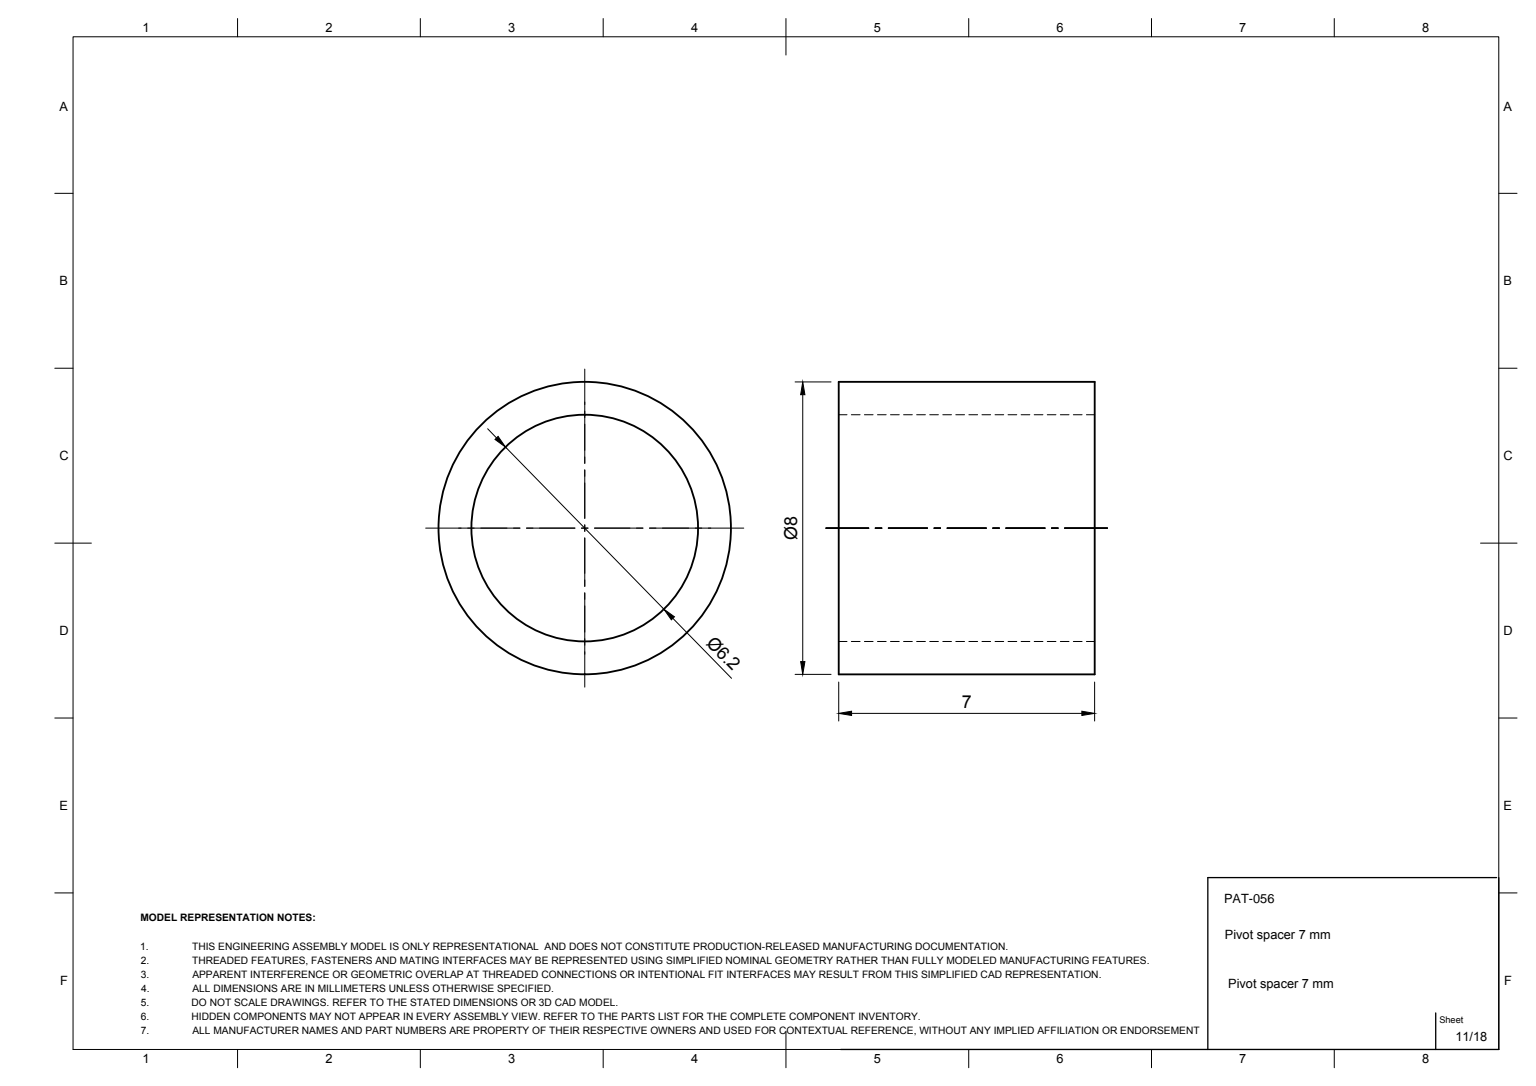
ISO-10303-21;
HEADER;
/* Generated by software containing ST-Developer
 * from STEP Tools, Inc. (www.steptools.com) 
 */

FILE_DESCRIPTION(
/* description */ ('Hook toggle clamp'),
/* implementation_level */ '2;1');

FILE_NAME(
/* name */ 'Pivot spacer 7 mm.step',
/* time_stamp */ '2026-10-27T21:56:56-07:00',
/* author */ (''),
/* organization */ (''),
/* preprocessor_version */ 'ST-DEVELOPER v20.2',
/* originating_system */ 'Autodesk Translation Framework v15.17.0.0',
/* authorisation */ '');

FILE_SCHEMA (('AUTOMOTIVE_DESIGN { 1 0 10303 214 3 1 1 }'));
ENDSEC;

DATA;
#10=MECHANICAL_DESIGN_GEOMETRIC_PRESENTATION_REPRESENTATION('',(#194),#5458);
#160=SHAPE_REPRESENTATION_RELATIONSHIP('SRR','None',#5542,#177);
#177=ADVANCED_BREP_SHAPE_REPRESENTATION('',(#211),#5444);
#194=STYLED_ITEM('',(#5703),#211);
#211=MANIFOLD_SOLID_BREP('Body1',#2975);
#251=FACE_BOUND('',#676,.T.);
#252=FACE_BOUND('',#678,.T.);
#336=PLANE('',#3312);
#337=PLANE('',#3313);
#471=FACE_OUTER_BOUND('',#673,.T.);
#472=FACE_OUTER_BOUND('',#674,.T.);
#473=FACE_OUTER_BOUND('',#675,.T.);
#474=FACE_OUTER_BOUND('',#677,.T.);
#673=EDGE_LOOP('',(#2377,#2378,#2379,#2380));
#674=EDGE_LOOP('',(#2381,#2382,#2383,#2384));
#675=EDGE_LOOP('',(#2385));
#676=EDGE_LOOP('',(#2386));
#677=EDGE_LOOP('',(#2387));
#678=EDGE_LOOP('',(#2388));
#934=LINE('',#4834,#1171);
#935=LINE('',#4840,#1172);
#1171=VECTOR('',#3914,0.31);
#1172=VECTOR('',#3921,0.4);
#1312=CIRCLE('',#3307,0.31);
#1313=CIRCLE('',#3308,0.31);
#1314=CIRCLE('',#3310,0.4);
#1315=CIRCLE('',#3311,0.4);
#1507=VERTEX_POINT('',#4831);
#1508=VERTEX_POINT('',#4833);
#1509=VERTEX_POINT('',#4837);
#1510=VERTEX_POINT('',#4839);
#1815=EDGE_CURVE('',#1507,#1507,#1312,.T.);
#1816=EDGE_CURVE('',#1507,#1508,#934,.T.);
#1817=EDGE_CURVE('',#1508,#1508,#1313,.T.);
#1818=EDGE_CURVE('',#1509,#1509,#1314,.T.);
#1819=EDGE_CURVE('',#1509,#1510,#935,.T.);
#1820=EDGE_CURVE('',#1510,#1510,#1315,.T.);
#2377=ORIENTED_EDGE('',*,*,#1815,.F.);
#2378=ORIENTED_EDGE('',*,*,#1816,.T.);
#2379=ORIENTED_EDGE('',*,*,#1817,.T.);
#2380=ORIENTED_EDGE('',*,*,#1816,.F.);
#2381=ORIENTED_EDGE('',*,*,#1818,.F.);
#2382=ORIENTED_EDGE('',*,*,#1819,.T.);
#2383=ORIENTED_EDGE('',*,*,#1820,.T.);
#2384=ORIENTED_EDGE('',*,*,#1819,.F.);
#2385=ORIENTED_EDGE('',*,*,#1818,.T.);
#2386=ORIENTED_EDGE('',*,*,#1815,.T.);
#2387=ORIENTED_EDGE('',*,*,#1820,.F.);
#2388=ORIENTED_EDGE('',*,*,#1817,.F.);
#2768=CYLINDRICAL_SURFACE('',#3306,0.31);
#2769=CYLINDRICAL_SURFACE('',#3309,0.4);
#2875=ADVANCED_FACE('',(#471),#2768,.F.);
#2876=ADVANCED_FACE('',(#472),#2769,.T.);
#2877=ADVANCED_FACE('',(#473,#251),#336,.T.);
#2878=ADVANCED_FACE('',(#474,#252),#337,.F.);
#2975=CLOSED_SHELL('',(#2875,#2876,#2877,#2878));
#3305=AXIS2_PLACEMENT_3D('',#4829,#3908,#3909);
#3306=AXIS2_PLACEMENT_3D('',#4830,#3910,#3911);
#3307=AXIS2_PLACEMENT_3D('',#4832,#3912,#3913);
#3308=AXIS2_PLACEMENT_3D('',#4835,#3915,#3916);
#3309=AXIS2_PLACEMENT_3D('',#4836,#3917,#3918);
#3310=AXIS2_PLACEMENT_3D('',#4838,#3919,#3920);
#3311=AXIS2_PLACEMENT_3D('',#4841,#3922,#3923);
#3312=AXIS2_PLACEMENT_3D('',#4842,#3924,#3925);
#3313=AXIS2_PLACEMENT_3D('',#4843,#3926,#3927);
#3908=DIRECTION('axis',(0.,0.,1.));
#3909=DIRECTION('refdir',(1.,0.,0.));
#3910=DIRECTION('center_axis',(0.,1.,0.));
#3911=DIRECTION('ref_axis',(1.,0.,0.));
#3912=DIRECTION('center_axis',(0.,-1.,0.));
#3913=DIRECTION('ref_axis',(1.,0.,0.));
#3914=DIRECTION('',(0.,-1.,0.));
#3915=DIRECTION('center_axis',(0.,-1.,0.));
#3916=DIRECTION('ref_axis',(1.,0.,0.));
#3917=DIRECTION('center_axis',(0.,1.,0.));
#3918=DIRECTION('ref_axis',(1.,0.,0.));
#3919=DIRECTION('center_axis',(0.,1.,0.));
#3920=DIRECTION('ref_axis',(1.,0.,0.));
#3921=DIRECTION('',(0.,-1.,0.));
#3922=DIRECTION('center_axis',(0.,1.,0.));
#3923=DIRECTION('ref_axis',(1.,0.,0.));
#3924=DIRECTION('center_axis',(0.,1.,0.));
#3925=DIRECTION('ref_axis',(1.,0.,0.));
#3926=DIRECTION('center_axis',(0.,1.,0.));
#3927=DIRECTION('ref_axis',(1.,0.,0.));
#4829=CARTESIAN_POINT('',(0.,0.,0.));
#4830=CARTESIAN_POINT('Origin',(-2.49048674522936,0.4,2.28211064313086));
#4831=CARTESIAN_POINT('',(-2.80048674522936,1.1,2.28211064313086));
#4832=CARTESIAN_POINT('Origin',(-2.49048674522936,1.1,2.28211064313086));
#4833=CARTESIAN_POINT('',(-2.80048674522936,0.4,2.28211064313086));
#4834=CARTESIAN_POINT('',(-2.80048674522936,0.4,2.28211064313086));
#4835=CARTESIAN_POINT('Origin',(-2.49048674522936,0.4,2.28211064313086));
#4836=CARTESIAN_POINT('Origin',(-2.49048674522936,0.4,2.28211064313086));
#4837=CARTESIAN_POINT('',(-2.89048674522936,1.1,2.28211064313086));
#4838=CARTESIAN_POINT('Origin',(-2.49048674522936,1.1,2.28211064313086));
#4839=CARTESIAN_POINT('',(-2.89048674522936,0.4,2.28211064313086));
#4840=CARTESIAN_POINT('',(-2.89048674522936,0.4,2.28211064313086));
#4841=CARTESIAN_POINT('Origin',(-2.49048674522936,0.4,2.28211064313086));
#4842=CARTESIAN_POINT('Origin',(-2.49048674522936,1.1,2.28211064313086));
#4843=CARTESIAN_POINT('Origin',(-2.49048674522936,0.4,2.28211064313086));
#5421=UNCERTAINTY_MEASURE_WITH_UNIT(LENGTH_MEASURE(0.001),#5459,
'DISTANCE_ACCURACY_VALUE',
'Maximum model space distance between geometric entities at asserted c
onnectivities');
#5435=UNCERTAINTY_MEASURE_WITH_UNIT(LENGTH_MEASURE(0.001),#5459,
'DISTANCE_ACCURACY_VALUE',
'Maximum model space distance between geometric entities at asserted c
onnectivities');
#5444=(
GEOMETRIC_REPRESENTATION_CONTEXT(3)
GLOBAL_UNCERTAINTY_ASSIGNED_CONTEXT((#5421))
GLOBAL_UNIT_ASSIGNED_CONTEXT((#5459,#5461,#5462))
REPRESENTATION_CONTEXT('','3D')
);
#5458=(
GEOMETRIC_REPRESENTATION_CONTEXT(3)
GLOBAL_UNCERTAINTY_ASSIGNED_CONTEXT((#5435))
GLOBAL_UNIT_ASSIGNED_CONTEXT((#5459,#5461,#5462))
REPRESENTATION_CONTEXT('','3D')
);
#5459=(
LENGTH_UNIT()
NAMED_UNIT(*)
SI_UNIT(.CENTI.,.METRE.)
);
#5461=(
NAMED_UNIT(*)
PLANE_ANGLE_UNIT()
SI_UNIT($,.RADIAN.)
);
#5462=(
NAMED_UNIT(*)
SI_UNIT($,.STERADIAN.)
SOLID_ANGLE_UNIT()
);
#5471=SHAPE_DEFINITION_REPRESENTATION(#5493,#5542);
#5493=PRODUCT_DEFINITION_SHAPE('',$,#5565);
#5542=SHAPE_REPRESENTATION('',(#3305),#5444);
#5556=PRODUCT_DEFINITION_CONTEXT('part definition',#5624,'design');
#5565=PRODUCT_DEFINITION('Pivot spacer 7 mm','Pivot spacer 7 mm',#5587,
#5556);
#5587=PRODUCT_DEFINITION_FORMATION('',$,#5634);
#5624=APPLICATION_CONTEXT(
'Core Data for Automotive Mechanical Design Process');
#5625=PRODUCT_CONTEXT('part definition',#5624,'mechanical');
#5634=PRODUCT('Pivot spacer 7 mm','Pivot spacer 7 mm',
'Pivot spacer 7 mm',(#5625));
#5697=COLOUR_RGB('Light Blue',0.38,0.62,0.78);
#5698=FILL_AREA_STYLE_COLOUR('',#5697);
#5699=FILL_AREA_STYLE('',(#5698));
#5700=SURFACE_STYLE_FILL_AREA(#5699);
#5701=SURFACE_SIDE_STYLE('',(#5700));
#5702=SURFACE_STYLE_USAGE(.BOTH.,#5701);
#5703=PRESENTATION_STYLE_ASSIGNMENT((#5702));
ENDSEC;
END-ISO-10303-21;
